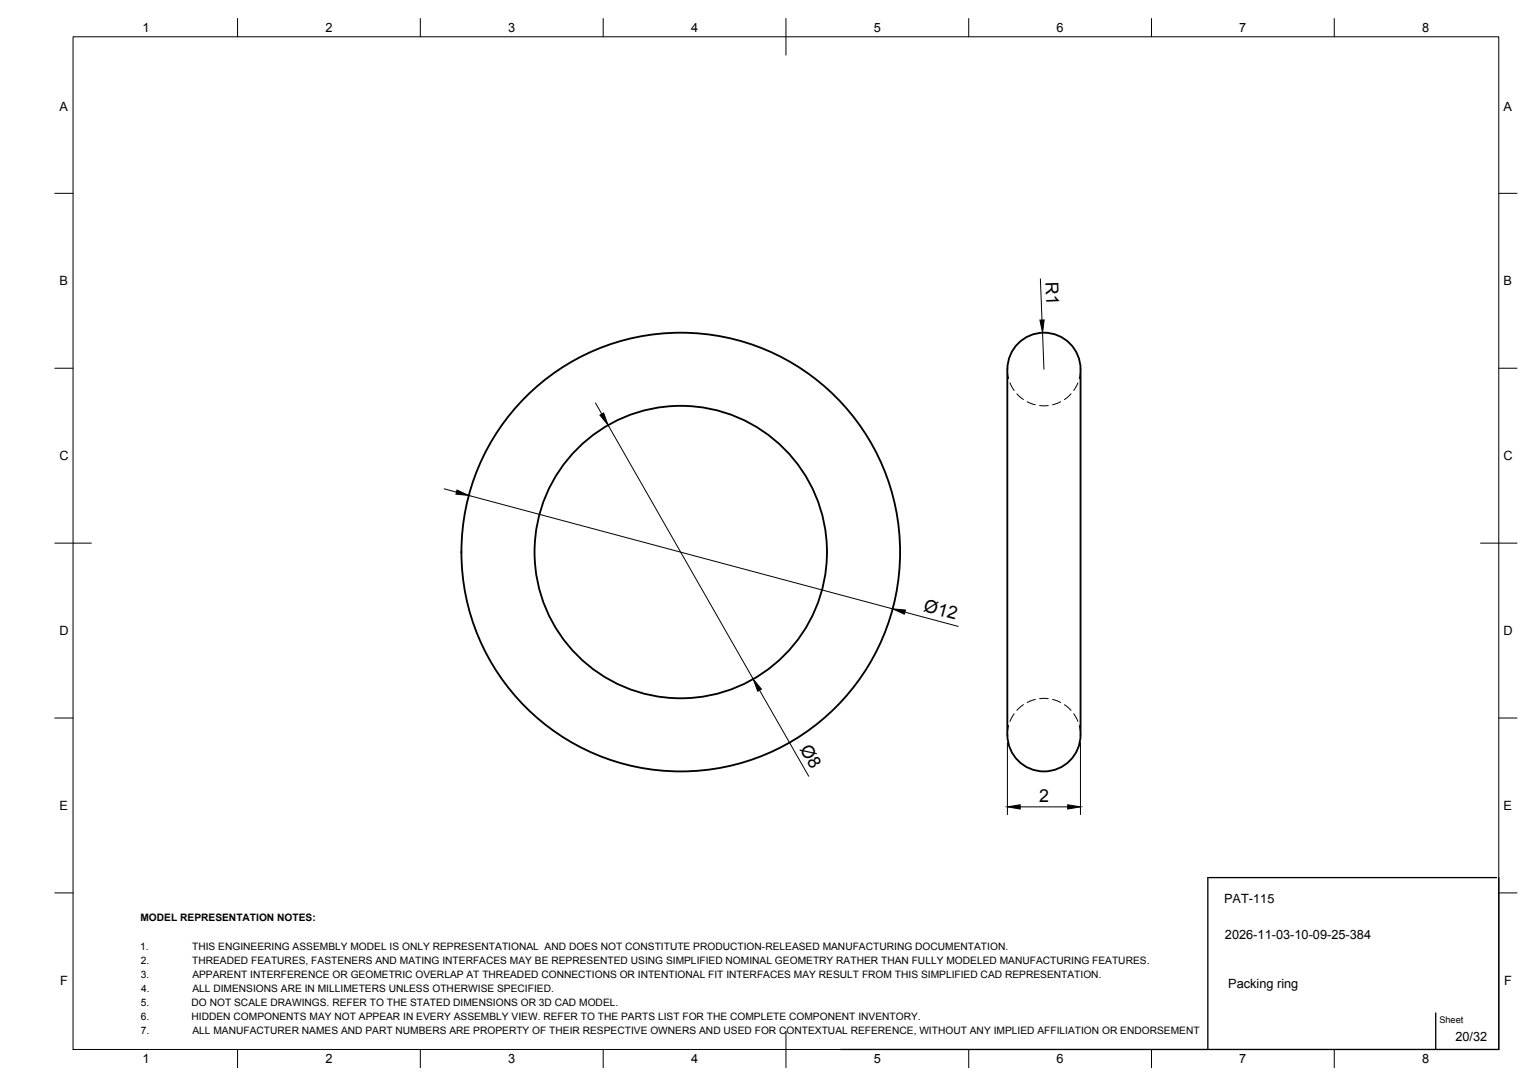
ISO-10303-21;
HEADER;
/* Generated by software containing ST-Developer
 * from STEP Tools, Inc. (www.steptools.com) 
 */

FILE_DESCRIPTION(
/* description */ ('Union bypass pipe loop'),
/* implementation_level */ '2;1');

FILE_NAME(
/* name */ 'Packing ring.step',
/* time_stamp */ '2026-10-27T21:00:29-07:00',
/* author */ (''),
/* organization */ (''),
/* preprocessor_version */ 'ST-DEVELOPER v20.2',
/* originating_system */ 'Autodesk Translation Framework v15.17.0.0',
/* authorisation */ '');

FILE_SCHEMA (('AUTOMOTIVE_DESIGN { 1 0 10303 214 3 1 1 }'));
ENDSEC;

DATA;
#10=MECHANICAL_DESIGN_GEOMETRIC_PRESENTATION_REPRESENTATION('',(#449),#10095);
#380=TOROIDAL_SURFACE('',#6035,0.5,0.1);
#385=SHAPE_REPRESENTATION_RELATIONSHIP('SRR','None',#10254,#417);
#417=ADVANCED_BREP_SHAPE_REPRESENTATION('',(#481),#10066);
#449=STYLED_ITEM('',(#10493),#481);
#481=MANIFOLD_SOLID_BREP('Body1',#5520);
#899=FACE_OUTER_BOUND('',#1270,.T.);
#1270=EDGE_LOOP('',(#4024,#4025,#4026,#4027));
#2433=CIRCLE('',#6036,0.1);
#2434=CIRCLE('',#6037,0.4);
#2726=VERTEX_POINT('',#8735);
#3210=EDGE_CURVE('',#2726,#2726,#2433,.T.);
#3211=EDGE_CURVE('',#2726,#2726,#2434,.T.);
#4024=ORIENTED_EDGE('',*,*,#3210,.F.);
#4025=ORIENTED_EDGE('',*,*,#3211,.T.);
#4026=ORIENTED_EDGE('',*,*,#3210,.T.);
#4027=ORIENTED_EDGE('',*,*,#3211,.F.);
#5248=ADVANCED_FACE('',(#899),#380,.T.);
#5520=CLOSED_SHELL('',(#5248));
#6034=AXIS2_PLACEMENT_3D('',#8733,#6962,#6963);
#6035=AXIS2_PLACEMENT_3D('',#8734,#6964,#6965);
#6036=AXIS2_PLACEMENT_3D('',#8736,#6966,#6967);
#6037=AXIS2_PLACEMENT_3D('',#8737,#6968,#6969);
#6962=DIRECTION('axis',(0.,0.,1.));
#6963=DIRECTION('refdir',(1.,0.,0.));
#6964=DIRECTION('center_axis',(0.,0.,1.));
#6965=DIRECTION('ref_axis',(1.,0.,0.));
#6966=DIRECTION('center_axis',(1.22464679914735E-16,-1.,0.));
#6967=DIRECTION('ref_axis',(-1.,-1.22464679914735E-16,0.));
#6968=DIRECTION('center_axis',(0.,0.,-1.));
#6969=DIRECTION('ref_axis',(1.,0.,0.));
#8733=CARTESIAN_POINT('',(0.,0.,0.));
#8734=CARTESIAN_POINT('Origin',(0.,0.,8.1));
#8735=CARTESIAN_POINT('',(-0.4,-4.89858719658941E-17,8.1));
#8736=CARTESIAN_POINT('Origin',(-0.5,-6.12323399573677E-17,8.1));
#8737=CARTESIAN_POINT('Origin',(0.,0.,8.1));
#10029=UNCERTAINTY_MEASURE_WITH_UNIT(LENGTH_MEASURE(0.001),#10096,
'DISTANCE_ACCURACY_VALUE',
'Maximum model space distance between geometric entities at asserted c
onnectivities');
#10058=UNCERTAINTY_MEASURE_WITH_UNIT(LENGTH_MEASURE(0.001),#10096,
'DISTANCE_ACCURACY_VALUE',
'Maximum model space distance between geometric entities at asserted c
onnectivities');
#10066=(
GEOMETRIC_REPRESENTATION_CONTEXT(3)
GLOBAL_UNCERTAINTY_ASSIGNED_CONTEXT((#10029))
GLOBAL_UNIT_ASSIGNED_CONTEXT((#10096,#10098,#10099))
REPRESENTATION_CONTEXT('','3D')
);
#10095=(
GEOMETRIC_REPRESENTATION_CONTEXT(3)
GLOBAL_UNCERTAINTY_ASSIGNED_CONTEXT((#10058))
GLOBAL_UNIT_ASSIGNED_CONTEXT((#10096,#10098,#10099))
REPRESENTATION_CONTEXT('','3D')
);
#10096=(
LENGTH_UNIT()
NAMED_UNIT(*)
SI_UNIT(.CENTI.,.METRE.)
);
#10098=(
NAMED_UNIT(*)
PLANE_ANGLE_UNIT()
SI_UNIT($,.RADIAN.)
);
#10099=(
NAMED_UNIT(*)
SI_UNIT($,.STERADIAN.)
SOLID_ANGLE_UNIT()
);
#10107=SHAPE_DEFINITION_REPRESENTATION(#10143,#10254);
#10143=PRODUCT_DEFINITION_SHAPE('',$,#10291);
#10254=SHAPE_REPRESENTATION('',(#6034),#10066);
#10283=PRODUCT_DEFINITION_CONTEXT('part definition',#10393,'design');
#10291=PRODUCT_DEFINITION('Packing ring','Packing ring',#10327,#10283);
#10327=PRODUCT_DEFINITION_FORMATION('',$,#10402);
#10393=APPLICATION_CONTEXT(
'Core Data for Automotive Mechanical Design Process');
#10394=PRODUCT_CONTEXT('part definition',#10393,'mechanical');
#10402=PRODUCT('Packing ring','Packing ring','Packing ring',(#10394));
#10487=COLOUR_RGB('Sky Blue',0.24,0.69,0.87);
#10488=FILL_AREA_STYLE_COLOUR('',#10487);
#10489=FILL_AREA_STYLE('',(#10488));
#10490=SURFACE_STYLE_FILL_AREA(#10489);
#10491=SURFACE_SIDE_STYLE('',(#10490));
#10492=SURFACE_STYLE_USAGE(.BOTH.,#10491);
#10493=PRESENTATION_STYLE_ASSIGNMENT((#10492));
ENDSEC;
END-ISO-10303-21;
